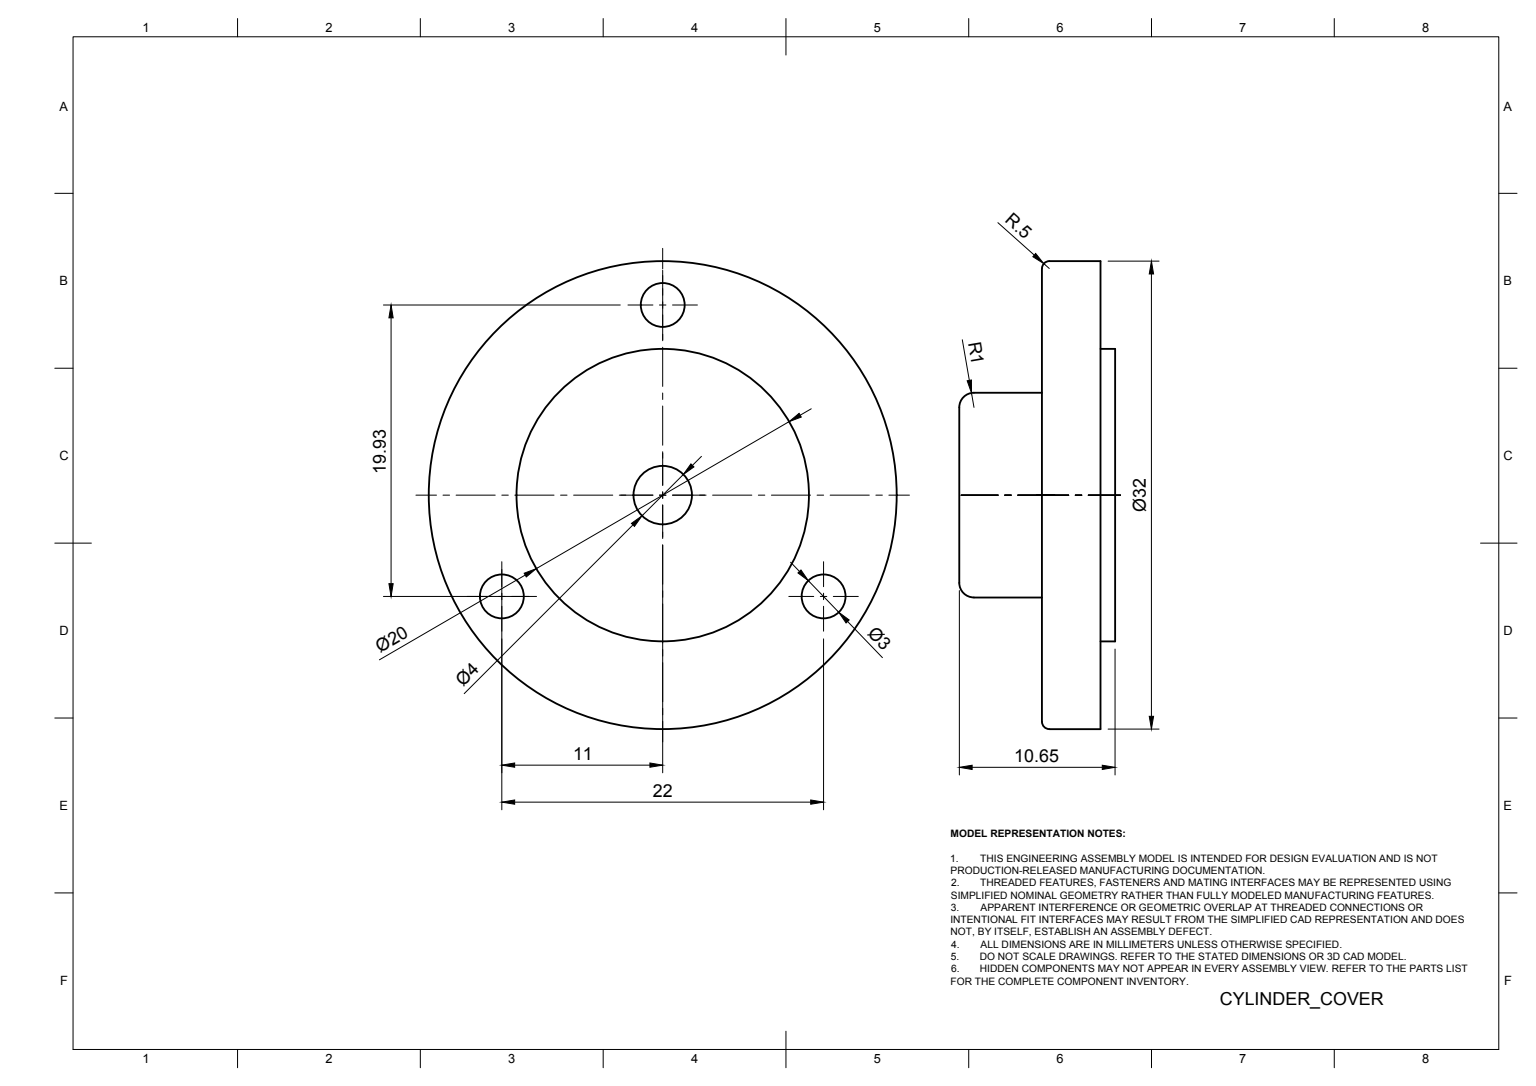
ISO-10303-21;
HEADER;
/* Generated by software containing ST-Developer
 * from STEP Tools, Inc. (www.steptools.com) 
 */

FILE_DESCRIPTION(
/* description */ (''),
/* implementation_level */ '2;1');

FILE_NAME(
/* name */ 'CYLINDERCOVER.step',
/* time_stamp */ '2026-10-06T01:16:10-07:00',
/* author */ (''),
/* organization */ (''),
/* preprocessor_version */ 'ST-DEVELOPER v20.2',
/* originating_system */ 'Autodesk Translation Framework v15.15.0.0',
/* authorisation */ '');

FILE_SCHEMA (('AUTOMOTIVE_DESIGN { 1 0 10303 214 3 1 1 }'));
ENDSEC;

DATA;
#10=MECHANICAL_DESIGN_GEOMETRIC_PRESENTATION_REPRESENTATION('',(#318),#17113);
#142=TOROIDAL_SURFACE('',#6796,6.,1.);
#143=TOROIDAL_SURFACE('',#6810,15.5,0.5);
#273=SHAPE_REPRESENTATION_RELATIONSHIP('SRR','None',#17198,#289);
#289=ADVANCED_BREP_SHAPE_REPRESENTATION('',(#339),#17105);
#318=STYLED_ITEM('',(#17298),#339);
#339=MANIFOLD_SOLID_BREP('Body1',#6025);
#466=CYLINDRICAL_SURFACE('',#6788,10.);
#467=CYLINDRICAL_SURFACE('',#6792,2.);
#468=CYLINDRICAL_SURFACE('',#6800,7.);
#469=CYLINDRICAL_SURFACE('',#6807,1.5);
#470=CYLINDRICAL_SURFACE('',#6808,1.5);
#471=CYLINDRICAL_SURFACE('',#6809,1.5);
#472=CYLINDRICAL_SURFACE('',#6814,16.);
#606=FACE_BOUND('',#1739,.T.);
#607=FACE_BOUND('',#1740,.T.);
#608=FACE_BOUND('',#1741,.T.);
#609=FACE_BOUND('',#1742,.T.);
#610=FACE_BOUND('',#1745,.T.);
#611=FACE_BOUND('',#1748,.T.);
#612=FACE_BOUND('',#1752,.T.);
#613=FACE_BOUND('',#1753,.T.);
#614=FACE_BOUND('',#1754,.T.);
#615=FACE_BOUND('',#1755,.T.);
#918=CIRCLE('',#6783,16.);
#919=CIRCLE('',#6784,10.);
#920=CIRCLE('',#6785,1.5);
#921=CIRCLE('',#6786,1.5);
#922=CIRCLE('',#6787,1.5);
#923=CIRCLE('',#6789,10.);
#924=CIRCLE('',#6791,2.);
#925=CIRCLE('',#6793,2.);
#926=CIRCLE('',#6795,6.);
#927=CIRCLE('',#6797,1.);
#928=CIRCLE('',#6798,7.);
#929=CIRCLE('',#6799,7.);
#930=CIRCLE('',#6801,7.);
#931=CIRCLE('',#6803,15.5);
#932=CIRCLE('',#6804,1.5);
#933=CIRCLE('',#6805,1.5);
#934=CIRCLE('',#6806,1.5);
#935=CIRCLE('',#6811,0.5);
#936=CIRCLE('',#6812,16.);
#937=CIRCLE('',#6813,16.);
#1276=FACE_OUTER_BOUND('',#1738,.T.);
#1277=FACE_OUTER_BOUND('',#1743,.T.);
#1278=FACE_OUTER_BOUND('',#1744,.T.);
#1279=FACE_OUTER_BOUND('',#1746,.T.);
#1280=FACE_OUTER_BOUND('',#1747,.T.);
#1281=FACE_OUTER_BOUND('',#1749,.T.);
#1282=FACE_OUTER_BOUND('',#1750,.T.);
#1283=FACE_OUTER_BOUND('',#1751,.T.);
#1284=FACE_OUTER_BOUND('',#1756,.T.);
#1285=FACE_OUTER_BOUND('',#1757,.T.);
#1286=FACE_OUTER_BOUND('',#1758,.T.);
#1287=FACE_OUTER_BOUND('',#1759,.T.);
#1288=FACE_OUTER_BOUND('',#1760,.T.);
#1738=EDGE_LOOP('',(#5122));
#1739=EDGE_LOOP('',(#5123));
#1740=EDGE_LOOP('',(#5124));
#1741=EDGE_LOOP('',(#5125));
#1742=EDGE_LOOP('',(#5126));
#1743=EDGE_LOOP('',(#5127,#5128,#5129,#5130));
#1744=EDGE_LOOP('',(#5131));
#1745=EDGE_LOOP('',(#5132));
#1746=EDGE_LOOP('',(#5133,#5134,#5135,#5136));
#1747=EDGE_LOOP('',(#5137));
#1748=EDGE_LOOP('',(#5138));
#1749=EDGE_LOOP('',(#5139,#5140,#5141,#5142,#5143));
#1750=EDGE_LOOP('',(#5144,#5145,#5146,#5147,#5148));
#1751=EDGE_LOOP('',(#5149));
#1752=EDGE_LOOP('',(#5150));
#1753=EDGE_LOOP('',(#5151));
#1754=EDGE_LOOP('',(#5152));
#1755=EDGE_LOOP('',(#5153));
#1756=EDGE_LOOP('',(#5154,#5155,#5156,#5157));
#1757=EDGE_LOOP('',(#5158,#5159,#5160,#5161));
#1758=EDGE_LOOP('',(#5162,#5163,#5164,#5165));
#1759=EDGE_LOOP('',(#5166,#5167,#5168,#5169,#5170));
#1760=EDGE_LOOP('',(#5171,#5172,#5173,#5174,#5175));
#2133=LINE('',#11477,#2494);
#2134=LINE('',#11484,#2495);
#2135=LINE('',#11497,#2496);
#2136=LINE('',#11509,#2497);
#2137=LINE('',#11511,#2498);
#2138=LINE('',#11513,#2499);
#2139=LINE('',#11521,#2500);
#2494=VECTOR('',#8411,10.);
#2495=VECTOR('',#8420,2.);
#2496=VECTOR('',#8437,7.);
#2497=VECTOR('',#8452,1.5);
#2498=VECTOR('',#8455,1.5);
#2499=VECTOR('',#8458,1.5);
#2500=VECTOR('',#8469,16.);
#2974=VERTEX_POINT('',#11465);
#2975=VERTEX_POINT('',#11467);
#2976=VERTEX_POINT('',#11469);
#2977=VERTEX_POINT('',#11471);
#2978=VERTEX_POINT('',#11473);
#2979=VERTEX_POINT('',#11476);
#2980=VERTEX_POINT('',#11480);
#2981=VERTEX_POINT('',#11483);
#2982=VERTEX_POINT('',#11487);
#2983=VERTEX_POINT('',#11490);
#2984=VERTEX_POINT('',#11492);
#2985=VERTEX_POINT('',#11496);
#2986=VERTEX_POINT('',#11500);
#2987=VERTEX_POINT('',#11502);
#2988=VERTEX_POINT('',#11504);
#2989=VERTEX_POINT('',#11506);
#2990=VERTEX_POINT('',#11515);
#2991=VERTEX_POINT('',#11517);
#3720=EDGE_CURVE('',#2974,#2974,#918,.T.);
#3721=EDGE_CURVE('',#2975,#2975,#919,.T.);
#3722=EDGE_CURVE('',#2976,#2976,#920,.T.);
#3723=EDGE_CURVE('',#2977,#2977,#921,.T.);
#3724=EDGE_CURVE('',#2978,#2978,#922,.T.);
#3725=EDGE_CURVE('',#2975,#2979,#2133,.T.);
#3726=EDGE_CURVE('',#2979,#2979,#923,.T.);
#3727=EDGE_CURVE('',#2980,#2980,#924,.T.);
#3728=EDGE_CURVE('',#2980,#2981,#2134,.T.);
#3729=EDGE_CURVE('',#2981,#2981,#925,.T.);
#3730=EDGE_CURVE('',#2982,#2982,#926,.T.);
#3731=EDGE_CURVE('',#2982,#2983,#927,.T.);
#3732=EDGE_CURVE('',#2983,#2984,#928,.T.);
#3733=EDGE_CURVE('',#2984,#2983,#929,.T.);
#3734=EDGE_CURVE('',#2984,#2985,#2135,.T.);
#3735=EDGE_CURVE('',#2985,#2985,#930,.T.);
#3736=EDGE_CURVE('',#2986,#2986,#931,.T.);
#3737=EDGE_CURVE('',#2987,#2987,#932,.T.);
#3738=EDGE_CURVE('',#2988,#2988,#933,.T.);
#3739=EDGE_CURVE('',#2989,#2989,#934,.T.);
#3740=EDGE_CURVE('',#2976,#2987,#2136,.T.);
#3741=EDGE_CURVE('',#2977,#2988,#2137,.T.);
#3742=EDGE_CURVE('',#2978,#2989,#2138,.T.);
#3743=EDGE_CURVE('',#2986,#2990,#935,.T.);
#3744=EDGE_CURVE('',#2990,#2991,#936,.T.);
#3745=EDGE_CURVE('',#2991,#2990,#937,.T.);
#3746=EDGE_CURVE('',#2991,#2974,#2139,.T.);
#5122=ORIENTED_EDGE('',*,*,#3720,.T.);
#5123=ORIENTED_EDGE('',*,*,#3721,.T.);
#5124=ORIENTED_EDGE('',*,*,#3722,.T.);
#5125=ORIENTED_EDGE('',*,*,#3723,.T.);
#5126=ORIENTED_EDGE('',*,*,#3724,.T.);
#5127=ORIENTED_EDGE('',*,*,#3721,.F.);
#5128=ORIENTED_EDGE('',*,*,#3725,.T.);
#5129=ORIENTED_EDGE('',*,*,#3726,.T.);
#5130=ORIENTED_EDGE('',*,*,#3725,.F.);
#5131=ORIENTED_EDGE('',*,*,#3726,.F.);
#5132=ORIENTED_EDGE('',*,*,#3727,.T.);
#5133=ORIENTED_EDGE('',*,*,#3727,.F.);
#5134=ORIENTED_EDGE('',*,*,#3728,.T.);
#5135=ORIENTED_EDGE('',*,*,#3729,.T.);
#5136=ORIENTED_EDGE('',*,*,#3728,.F.);
#5137=ORIENTED_EDGE('',*,*,#3730,.T.);
#5138=ORIENTED_EDGE('',*,*,#3729,.F.);
#5139=ORIENTED_EDGE('',*,*,#3730,.F.);
#5140=ORIENTED_EDGE('',*,*,#3731,.T.);
#5141=ORIENTED_EDGE('',*,*,#3732,.T.);
#5142=ORIENTED_EDGE('',*,*,#3733,.T.);
#5143=ORIENTED_EDGE('',*,*,#3731,.F.);
#5144=ORIENTED_EDGE('',*,*,#3733,.F.);
#5145=ORIENTED_EDGE('',*,*,#3734,.T.);
#5146=ORIENTED_EDGE('',*,*,#3735,.F.);
#5147=ORIENTED_EDGE('',*,*,#3734,.F.);
#5148=ORIENTED_EDGE('',*,*,#3732,.F.);
#5149=ORIENTED_EDGE('',*,*,#3736,.T.);
#5150=ORIENTED_EDGE('',*,*,#3737,.F.);
#5151=ORIENTED_EDGE('',*,*,#3738,.F.);
#5152=ORIENTED_EDGE('',*,*,#3739,.F.);
#5153=ORIENTED_EDGE('',*,*,#3735,.T.);
#5154=ORIENTED_EDGE('',*,*,#3722,.F.);
#5155=ORIENTED_EDGE('',*,*,#3740,.T.);
#5156=ORIENTED_EDGE('',*,*,#3737,.T.);
#5157=ORIENTED_EDGE('',*,*,#3740,.F.);
#5158=ORIENTED_EDGE('',*,*,#3723,.F.);
#5159=ORIENTED_EDGE('',*,*,#3741,.T.);
#5160=ORIENTED_EDGE('',*,*,#3738,.T.);
#5161=ORIENTED_EDGE('',*,*,#3741,.F.);
#5162=ORIENTED_EDGE('',*,*,#3724,.F.);
#5163=ORIENTED_EDGE('',*,*,#3742,.T.);
#5164=ORIENTED_EDGE('',*,*,#3739,.T.);
#5165=ORIENTED_EDGE('',*,*,#3742,.F.);
#5166=ORIENTED_EDGE('',*,*,#3736,.F.);
#5167=ORIENTED_EDGE('',*,*,#3743,.T.);
#5168=ORIENTED_EDGE('',*,*,#3744,.T.);
#5169=ORIENTED_EDGE('',*,*,#3745,.T.);
#5170=ORIENTED_EDGE('',*,*,#3743,.F.);
#5171=ORIENTED_EDGE('',*,*,#3745,.F.);
#5172=ORIENTED_EDGE('',*,*,#3746,.T.);
#5173=ORIENTED_EDGE('',*,*,#3720,.F.);
#5174=ORIENTED_EDGE('',*,*,#3746,.F.);
#5175=ORIENTED_EDGE('',*,*,#3744,.F.);
#5612=PLANE('',#6782);
#5613=PLANE('',#6790);
#5614=PLANE('',#6794);
#5615=PLANE('',#6802);
#5924=ADVANCED_FACE('',(#1276,#606,#607,#608,#609),#5612,.F.);
#5925=ADVANCED_FACE('',(#1277),#466,.T.);
#5926=ADVANCED_FACE('',(#1278,#610),#5613,.F.);
#5927=ADVANCED_FACE('',(#1279),#467,.F.);
#5928=ADVANCED_FACE('',(#1280,#611),#5614,.T.);
#5929=ADVANCED_FACE('',(#1281),#142,.T.);
#5930=ADVANCED_FACE('',(#1282),#468,.T.);
#5931=ADVANCED_FACE('',(#1283,#612,#613,#614,#615),#5615,.T.);
#5932=ADVANCED_FACE('',(#1284),#469,.F.);
#5933=ADVANCED_FACE('',(#1285),#470,.F.);
#5934=ADVANCED_FACE('',(#1286),#471,.F.);
#5935=ADVANCED_FACE('',(#1287),#143,.T.);
#5936=ADVANCED_FACE('',(#1288),#472,.T.);
#6025=CLOSED_SHELL('',(#5924,#5925,#5926,#5927,#5928,#5929,#5930,#5931,
#5932,#5933,#5934,#5935,#5936));
#6781=AXIS2_PLACEMENT_3D('',#11463,#8395,#8396);
#6782=AXIS2_PLACEMENT_3D('',#11464,#8397,#8398);
#6783=AXIS2_PLACEMENT_3D('',#11466,#8399,#8400);
#6784=AXIS2_PLACEMENT_3D('',#11468,#8401,#8402);
#6785=AXIS2_PLACEMENT_3D('',#11470,#8403,#8404);
#6786=AXIS2_PLACEMENT_3D('',#11472,#8405,#8406);
#6787=AXIS2_PLACEMENT_3D('',#11474,#8407,#8408);
#6788=AXIS2_PLACEMENT_3D('',#11475,#8409,#8410);
#6789=AXIS2_PLACEMENT_3D('',#11478,#8412,#8413);
#6790=AXIS2_PLACEMENT_3D('',#11479,#8414,#8415);
#6791=AXIS2_PLACEMENT_3D('',#11481,#8416,#8417);
#6792=AXIS2_PLACEMENT_3D('',#11482,#8418,#8419);
#6793=AXIS2_PLACEMENT_3D('',#11485,#8421,#8422);
#6794=AXIS2_PLACEMENT_3D('',#11486,#8423,#8424);
#6795=AXIS2_PLACEMENT_3D('',#11488,#8425,#8426);
#6796=AXIS2_PLACEMENT_3D('',#11489,#8427,#8428);
#6797=AXIS2_PLACEMENT_3D('',#11491,#8429,#8430);
#6798=AXIS2_PLACEMENT_3D('',#11493,#8431,#8432);
#6799=AXIS2_PLACEMENT_3D('',#11494,#8433,#8434);
#6800=AXIS2_PLACEMENT_3D('',#11495,#8435,#8436);
#6801=AXIS2_PLACEMENT_3D('',#11498,#8438,#8439);
#6802=AXIS2_PLACEMENT_3D('',#11499,#8440,#8441);
#6803=AXIS2_PLACEMENT_3D('',#11501,#8442,#8443);
#6804=AXIS2_PLACEMENT_3D('',#11503,#8444,#8445);
#6805=AXIS2_PLACEMENT_3D('',#11505,#8446,#8447);
#6806=AXIS2_PLACEMENT_3D('',#11507,#8448,#8449);
#6807=AXIS2_PLACEMENT_3D('',#11508,#8450,#8451);
#6808=AXIS2_PLACEMENT_3D('',#11510,#8453,#8454);
#6809=AXIS2_PLACEMENT_3D('',#11512,#8456,#8457);
#6810=AXIS2_PLACEMENT_3D('',#11514,#8459,#8460);
#6811=AXIS2_PLACEMENT_3D('',#11516,#8461,#8462);
#6812=AXIS2_PLACEMENT_3D('',#11518,#8463,#8464);
#6813=AXIS2_PLACEMENT_3D('',#11519,#8465,#8466);
#6814=AXIS2_PLACEMENT_3D('',#11520,#8467,#8468);
#8395=DIRECTION('axis',(0.,0.,1.));
#8396=DIRECTION('refdir',(1.,0.,0.));
#8397=DIRECTION('center_axis',(0.,1.,0.));
#8398=DIRECTION('ref_axis',(1.,0.,0.));
#8399=DIRECTION('center_axis',(0.,-1.,0.));
#8400=DIRECTION('ref_axis',(1.,0.,0.));
#8401=DIRECTION('center_axis',(0.,1.,0.));
#8402=DIRECTION('ref_axis',(1.,0.,0.));
#8403=DIRECTION('center_axis',(0.,1.,0.));
#8404=DIRECTION('ref_axis',(1.,0.,0.));
#8405=DIRECTION('center_axis',(0.,1.,0.));
#8406=DIRECTION('ref_axis',(1.,0.,0.));
#8407=DIRECTION('center_axis',(0.,1.,0.));
#8408=DIRECTION('ref_axis',(1.,0.,0.));
#8409=DIRECTION('center_axis',(0.,1.,0.));
#8410=DIRECTION('ref_axis',(1.,0.,0.));
#8411=DIRECTION('',(0.,-1.,0.));
#8412=DIRECTION('center_axis',(0.,1.,0.));
#8413=DIRECTION('ref_axis',(1.,0.,0.));
#8414=DIRECTION('center_axis',(0.,1.,0.));
#8415=DIRECTION('ref_axis',(1.,0.,0.));
#8416=DIRECTION('center_axis',(0.,1.,0.));
#8417=DIRECTION('ref_axis',(1.,0.,0.));
#8418=DIRECTION('center_axis',(0.,1.,0.));
#8419=DIRECTION('ref_axis',(1.,0.,0.));
#8420=DIRECTION('',(0.,1.,0.));
#8421=DIRECTION('center_axis',(0.,1.,0.));
#8422=DIRECTION('ref_axis',(1.,0.,0.));
#8423=DIRECTION('center_axis',(0.,1.,0.));
#8424=DIRECTION('ref_axis',(1.,0.,0.));
#8425=DIRECTION('center_axis',(0.,1.,0.));
#8426=DIRECTION('ref_axis',(1.,0.,0.));
#8427=DIRECTION('center_axis',(0.,1.,0.));
#8428=DIRECTION('ref_axis',(0.999758738295459,0.,0.0219650905273091));
#8429=DIRECTION('center_axis',(-0.021965090527309,0.,0.999758738295459));
#8430=DIRECTION('ref_axis',(-0.999758738295459,0.,-0.021965090527309));
#8431=DIRECTION('center_axis',(0.,1.,0.));
#8432=DIRECTION('ref_axis',(1.,0.,0.));
#8433=DIRECTION('center_axis',(0.,1.,0.));
#8434=DIRECTION('ref_axis',(1.,0.,0.));
#8435=DIRECTION('center_axis',(0.,1.,0.));
#8436=DIRECTION('ref_axis',(1.,0.,0.));
#8437=DIRECTION('',(0.,-1.,0.));
#8438=DIRECTION('center_axis',(0.,-1.,0.));
#8439=DIRECTION('ref_axis',(1.,0.,0.));
#8440=DIRECTION('center_axis',(0.,1.,0.));
#8441=DIRECTION('ref_axis',(1.,0.,0.));
#8442=DIRECTION('center_axis',(0.,1.,0.));
#8443=DIRECTION('ref_axis',(1.,0.,0.));
#8444=DIRECTION('center_axis',(0.,1.,0.));
#8445=DIRECTION('ref_axis',(1.,0.,0.));
#8446=DIRECTION('center_axis',(0.,1.,0.));
#8447=DIRECTION('ref_axis',(1.,0.,0.));
#8448=DIRECTION('center_axis',(0.,1.,0.));
#8449=DIRECTION('ref_axis',(1.,0.,0.));
#8450=DIRECTION('center_axis',(0.,1.,0.));
#8451=DIRECTION('ref_axis',(1.,0.,0.));
#8452=DIRECTION('',(0.,1.,0.));
#8453=DIRECTION('center_axis',(0.,1.,0.));
#8454=DIRECTION('ref_axis',(1.,0.,0.));
#8455=DIRECTION('',(0.,1.,0.));
#8456=DIRECTION('center_axis',(0.,1.,0.));
#8457=DIRECTION('ref_axis',(1.,0.,0.));
#8458=DIRECTION('',(0.,1.,0.));
#8459=DIRECTION('center_axis',(0.,1.,0.));
#8460=DIRECTION('ref_axis',(0.999953819500319,0.,0.00961035206031418));
#8461=DIRECTION('center_axis',(-0.00961035206031406,0.,0.999953819500319));
#8462=DIRECTION('ref_axis',(-0.999953819500319,0.,-0.00961035206031406));
#8463=DIRECTION('center_axis',(0.,1.,0.));
#8464=DIRECTION('ref_axis',(1.,0.,0.));
#8465=DIRECTION('center_axis',(0.,1.,0.));
#8466=DIRECTION('ref_axis',(1.,0.,0.));
#8467=DIRECTION('center_axis',(0.,1.,0.));
#8468=DIRECTION('ref_axis',(1.,0.,0.));
#8469=DIRECTION('',(0.,-1.,0.));
#11463=CARTESIAN_POINT('',(0.,0.,0.));
#11464=CARTESIAN_POINT('Origin',(0.,0.,0.));
#11465=CARTESIAN_POINT('',(-16.,0.,1.95943487863577E-15));
#11466=CARTESIAN_POINT('Origin',(0.,0.,0.));
#11467=CARTESIAN_POINT('',(-10.,0.,0.));
#11468=CARTESIAN_POINT('Origin',(0.,0.,0.));
#11469=CARTESIAN_POINT('',(-14.5,0.,0.));
#11470=CARTESIAN_POINT('Origin',(-13.,0.,0.));
#11471=CARTESIAN_POINT('',(5.428203230276,0.,-11.));
#11472=CARTESIAN_POINT('Origin',(6.928203230276,0.,-11.));
#11473=CARTESIAN_POINT('',(5.428203230276,0.,11.));
#11474=CARTESIAN_POINT('Origin',(6.928203230276,0.,11.));
#11475=CARTESIAN_POINT('Origin',(0.,-1.5325,0.));
#11476=CARTESIAN_POINT('',(-10.,-1.,0.));
#11477=CARTESIAN_POINT('',(-10.,-1.5325,1.22464679914735E-15));
#11478=CARTESIAN_POINT('Origin',(0.,-1.,0.));
#11479=CARTESIAN_POINT('Origin',(0.,-1.,0.));
#11480=CARTESIAN_POINT('',(-2.,-1.,0.));
#11481=CARTESIAN_POINT('Origin',(0.,-1.,0.));
#11482=CARTESIAN_POINT('Origin',(0.,-1.5325,0.));
#11483=CARTESIAN_POINT('',(-2.,9.65,0.));
#11484=CARTESIAN_POINT('',(-2.,-1.5325,2.44929359829471E-16));
#11485=CARTESIAN_POINT('Origin',(0.,9.65,0.));
#11486=CARTESIAN_POINT('Origin',(0.,9.65,0.));
#11487=CARTESIAN_POINT('',(-5.99855242977275,9.65,-0.131790543163854));
#11488=CARTESIAN_POINT('Origin',(0.,9.65,0.));
#11489=CARTESIAN_POINT('Origin',(0.,8.65,0.));
#11490=CARTESIAN_POINT('',(-6.99831116806821,8.65,-0.153755633691163));
#11491=CARTESIAN_POINT('Origin',(-5.99855242977275,8.65,-0.131790543163854));
#11492=CARTESIAN_POINT('',(-7.,8.65,0.));
#11493=CARTESIAN_POINT('Origin',(0.,8.65,0.));
#11494=CARTESIAN_POINT('Origin',(0.,8.65,0.));
#11495=CARTESIAN_POINT('Origin',(0.,-1.5325,0.));
#11496=CARTESIAN_POINT('',(-7.,4.,8.57252759403147E-16));
#11497=CARTESIAN_POINT('',(-7.,-1.5325,8.57252759403147E-16));
#11498=CARTESIAN_POINT('Origin',(0.,4.,0.));
#11499=CARTESIAN_POINT('Origin',(0.,4.,0.));
#11500=CARTESIAN_POINT('',(-15.4992842022549,4.,-0.148960456934868));
#11501=CARTESIAN_POINT('Origin',(0.,4.,0.));
#11502=CARTESIAN_POINT('',(-14.5,4.,0.));
#11503=CARTESIAN_POINT('Origin',(-13.,4.,0.));
#11504=CARTESIAN_POINT('',(5.428203230276,4.,-11.));
#11505=CARTESIAN_POINT('Origin',(6.928203230276,4.,-11.));
#11506=CARTESIAN_POINT('',(5.428203230276,4.,11.));
#11507=CARTESIAN_POINT('Origin',(6.928203230276,4.,11.));
#11508=CARTESIAN_POINT('Origin',(-13.,4.,0.));
#11509=CARTESIAN_POINT('',(-14.5,4.,1.83697019872103E-16));
#11510=CARTESIAN_POINT('Origin',(6.928203230276,4.,-11.));
#11511=CARTESIAN_POINT('',(5.428203230276,4.,-11.));
#11512=CARTESIAN_POINT('Origin',(6.928203230276,4.,11.));
#11513=CARTESIAN_POINT('',(5.428203230276,4.,11.));
#11514=CARTESIAN_POINT('Origin',(0.,3.5,0.));
#11515=CARTESIAN_POINT('',(-15.9992611120051,3.5,-0.153765632965025));
#11516=CARTESIAN_POINT('Origin',(-15.4992842022549,3.5,-0.148960456934868));
#11517=CARTESIAN_POINT('',(-16.,3.5,0.));
#11518=CARTESIAN_POINT('Origin',(0.,3.5,0.));
#11519=CARTESIAN_POINT('Origin',(0.,3.5,0.));
#11520=CARTESIAN_POINT('Origin',(0.,-1.5325,0.));
#11521=CARTESIAN_POINT('',(-16.,-1.5325,1.95943487863577E-15));
#17082=UNCERTAINTY_MEASURE_WITH_UNIT(LENGTH_MEASURE(0.01),#17114,
'DISTANCE_ACCURACY_VALUE',
'Maximum model space distance between geometric entities at asserted c
onnectivities');
#17090=UNCERTAINTY_MEASURE_WITH_UNIT(LENGTH_MEASURE(0.01),#17114,
'DISTANCE_ACCURACY_VALUE',
'Maximum model space distance between geometric entities at asserted c
onnectivities');
#17105=(
GEOMETRIC_REPRESENTATION_CONTEXT(3)
GLOBAL_UNCERTAINTY_ASSIGNED_CONTEXT((#17082))
GLOBAL_UNIT_ASSIGNED_CONTEXT((#17114,#17116,#17117))
REPRESENTATION_CONTEXT('','3D')
);
#17113=(
GEOMETRIC_REPRESENTATION_CONTEXT(3)
GLOBAL_UNCERTAINTY_ASSIGNED_CONTEXT((#17090))
GLOBAL_UNIT_ASSIGNED_CONTEXT((#17114,#17116,#17117))
REPRESENTATION_CONTEXT('','3D')
);
#17114=(
LENGTH_UNIT()
NAMED_UNIT(*)
SI_UNIT(.MILLI.,.METRE.)
);
#17116=(
NAMED_UNIT(*)
PLANE_ANGLE_UNIT()
SI_UNIT($,.RADIAN.)
);
#17117=(
NAMED_UNIT(*)
SI_UNIT($,.STERADIAN.)
SOLID_ANGLE_UNIT()
);
#17132=SHAPE_DEFINITION_REPRESENTATION(#17163,#17198);
#17163=PRODUCT_DEFINITION_SHAPE('',$,#17221);
#17198=SHAPE_REPRESENTATION('',(#6781),#17105);
#17206=PRODUCT_DEFINITION_CONTEXT('part definition',#17274,'design');
#17221=PRODUCT_DEFINITION('CYLINDERCOVER','CYLINDERCOVER',#17243,#17206);
#17243=PRODUCT_DEFINITION_FORMATION('',$,#17290);
#17274=APPLICATION_CONTEXT(
'Core Data for Automotive Mechanical Design Process');
#17275=PRODUCT_CONTEXT('part definition',#17274,'mechanical');
#17290=PRODUCT('CYLINDERCOVER','CYLINDERCOVER','NOT SPECIFIED',(#17275));
#17298=PRESENTATION_STYLE_ASSIGNMENT((#17299));
#17299=SURFACE_STYLE_USAGE(.BOTH.,#17300);
#17300=SURFACE_SIDE_STYLE('',(#17301));
#17301=SURFACE_STYLE_FILL_AREA(#17302);
#17302=FILL_AREA_STYLE('Steel - Satin',(#17303));
#17303=FILL_AREA_STYLE_COLOUR('Steel - Satin',#17304);
#17304=COLOUR_RGB('Steel - Satin', 0.09019608, 0.27058824, 0.51372549);
ENDSEC;
END-ISO-10303-21;
